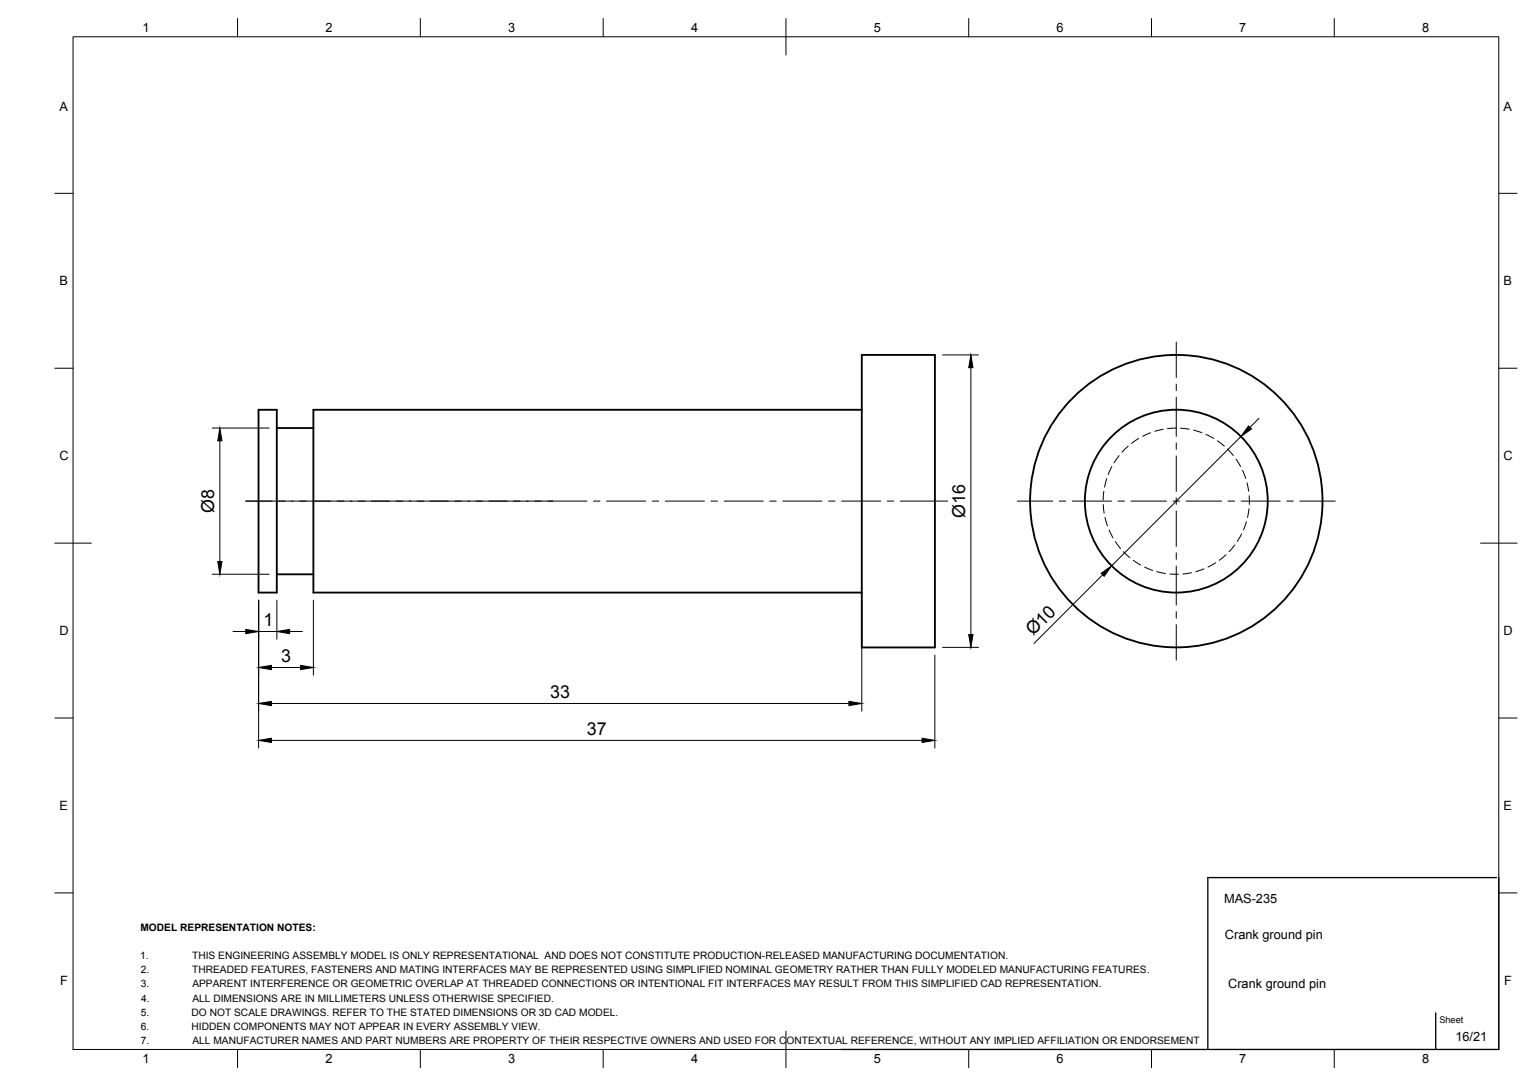
ISO-10303-21;
HEADER;
/* Generated by software containing ST-Developer
 * from STEP Tools, Inc. (www.steptools.com) 
 */

FILE_DESCRIPTION(
/* description */ ('Independent Whitworth quick-return mechanism. Crank radius40, ground-
center spacing80, lever180, connecting rod160, output guide X200. Nomi
nal stroke180 and long/short phase ratio2. Retained guide rods, replac
eable bearing sleeves and captured sliding shoe. No load or production
 rating assigned.'),
/* implementation_level */ '2;1');

FILE_NAME(
/* name */ 'Crank ground pin.step',
/* time_stamp */ '2026-11-09T18:22:56-08:00',
/* author */ (''),
/* organization */ (''),
/* preprocessor_version */ 'ST-DEVELOPER v20.2',
/* originating_system */ 'Autodesk Translation Framework v15.17.0.0',
/* authorisation */ '');

FILE_SCHEMA (('AUTOMOTIVE_DESIGN { 1 0 10303 214 3 1 1 }'));
ENDSEC;

DATA;
#10=MECHANICAL_DESIGN_GEOMETRIC_PRESENTATION_REPRESENTATION('',(#230),#4388);
#190=SHAPE_REPRESENTATION_RELATIONSHIP('SRR','None',#4489,#210);
#210=ADVANCED_BREP_SHAPE_REPRESENTATION('',(#250),#4379);
#230=STYLED_ITEM('',(#4595),#250);
#250=MANIFOLD_SOLID_BREP('Body1',#2335);
#296=FACE_BOUND('',#671,.T.);
#297=FACE_BOUND('',#673,.T.);
#298=FACE_BOUND('',#676,.T.);
#368=PLANE('',#2723);
#369=PLANE('',#2725);
#370=PLANE('',#2729);
#371=PLANE('',#2734);
#372=PLANE('',#2736);
#485=FACE_OUTER_BOUND('',#669,.T.);
#486=FACE_OUTER_BOUND('',#670,.T.);
#487=FACE_OUTER_BOUND('',#672,.T.);
#488=FACE_OUTER_BOUND('',#674,.T.);
#489=FACE_OUTER_BOUND('',#675,.T.);
#490=FACE_OUTER_BOUND('',#677,.T.);
#491=FACE_OUTER_BOUND('',#678,.T.);
#492=FACE_OUTER_BOUND('',#679,.T.);
#493=FACE_OUTER_BOUND('',#680,.T.);
#669=EDGE_LOOP('',(#1924,#1925,#1926,#1927));
#670=EDGE_LOOP('',(#1928));
#671=EDGE_LOOP('',(#1929));
#672=EDGE_LOOP('',(#1930));
#673=EDGE_LOOP('',(#1931));
#674=EDGE_LOOP('',(#1932,#1933,#1934,#1935));
#675=EDGE_LOOP('',(#1936));
#676=EDGE_LOOP('',(#1937));
#677=EDGE_LOOP('',(#1938,#1939,#1940,#1941));
#678=EDGE_LOOP('',(#1942));
#679=EDGE_LOOP('',(#1943,#1944,#1945,#1946));
#680=EDGE_LOOP('',(#1947));
#862=LINE('',#4072,#1001);
#863=LINE('',#4083,#1002);
#864=LINE('',#4091,#1003);
#865=LINE('',#4095,#1004);
#1001=VECTOR('',#3314,4.);
#1002=VECTOR('',#3329,5.);
#1003=VECTOR('',#3338,8.);
#1004=VECTOR('',#3345,5.);
#1099=CIRCLE('',#2721,4.);
#1100=CIRCLE('',#2722,4.);
#1101=CIRCLE('',#2724,5.);
#1102=CIRCLE('',#2726,5.);
#1103=CIRCLE('',#2728,5.);
#1104=CIRCLE('',#2730,8.);
#1105=CIRCLE('',#2731,5.);
#1106=CIRCLE('',#2733,8.);
#1269=VERTEX_POINT('',#4069);
#1270=VERTEX_POINT('',#4071);
#1271=VERTEX_POINT('',#4075);
#1272=VERTEX_POINT('',#4078);
#1273=VERTEX_POINT('',#4081);
#1274=VERTEX_POINT('',#4085);
#1275=VERTEX_POINT('',#4087);
#1276=VERTEX_POINT('',#4090);
#1498=EDGE_CURVE('',#1269,#1269,#1099,.T.);
#1499=EDGE_CURVE('',#1269,#1270,#862,.T.);
#1500=EDGE_CURVE('',#1270,#1270,#1100,.T.);
#1501=EDGE_CURVE('',#1271,#1271,#1101,.T.);
#1502=EDGE_CURVE('',#1272,#1272,#1102,.T.);
#1503=EDGE_CURVE('',#1273,#1273,#1103,.T.);
#1504=EDGE_CURVE('',#1273,#1272,#863,.T.);
#1505=EDGE_CURVE('',#1274,#1274,#1104,.T.);
#1506=EDGE_CURVE('',#1275,#1275,#1105,.T.);
#1507=EDGE_CURVE('',#1274,#1276,#864,.T.);
#1508=EDGE_CURVE('',#1276,#1276,#1106,.T.);
#1509=EDGE_CURVE('',#1271,#1275,#865,.T.);
#1924=ORIENTED_EDGE('',*,*,#1498,.T.);
#1925=ORIENTED_EDGE('',*,*,#1499,.T.);
#1926=ORIENTED_EDGE('',*,*,#1500,.F.);
#1927=ORIENTED_EDGE('',*,*,#1499,.F.);
#1928=ORIENTED_EDGE('',*,*,#1501,.F.);
#1929=ORIENTED_EDGE('',*,*,#1498,.F.);
#1930=ORIENTED_EDGE('',*,*,#1502,.F.);
#1931=ORIENTED_EDGE('',*,*,#1500,.T.);
#1932=ORIENTED_EDGE('',*,*,#1503,.F.);
#1933=ORIENTED_EDGE('',*,*,#1504,.T.);
#1934=ORIENTED_EDGE('',*,*,#1502,.T.);
#1935=ORIENTED_EDGE('',*,*,#1504,.F.);
#1936=ORIENTED_EDGE('',*,*,#1505,.T.);
#1937=ORIENTED_EDGE('',*,*,#1506,.F.);
#1938=ORIENTED_EDGE('',*,*,#1505,.F.);
#1939=ORIENTED_EDGE('',*,*,#1507,.T.);
#1940=ORIENTED_EDGE('',*,*,#1508,.T.);
#1941=ORIENTED_EDGE('',*,*,#1507,.F.);
#1942=ORIENTED_EDGE('',*,*,#1508,.F.);
#1943=ORIENTED_EDGE('',*,*,#1501,.T.);
#1944=ORIENTED_EDGE('',*,*,#1509,.T.);
#1945=ORIENTED_EDGE('',*,*,#1506,.T.);
#1946=ORIENTED_EDGE('',*,*,#1509,.F.);
#1947=ORIENTED_EDGE('',*,*,#1503,.T.);
#2147=CYLINDRICAL_SURFACE('',#2720,4.);
#2148=CYLINDRICAL_SURFACE('',#2727,5.);
#2149=CYLINDRICAL_SURFACE('',#2732,8.);
#2150=CYLINDRICAL_SURFACE('',#2735,5.);
#2257=ADVANCED_FACE('',(#485),#2147,.T.);
#2258=ADVANCED_FACE('',(#486,#296),#368,.F.);
#2259=ADVANCED_FACE('',(#487,#297),#369,.F.);
#2260=ADVANCED_FACE('',(#488),#2148,.T.);
#2261=ADVANCED_FACE('',(#489,#298),#370,.T.);
#2262=ADVANCED_FACE('',(#490),#2149,.T.);
#2263=ADVANCED_FACE('',(#491),#371,.F.);
#2264=ADVANCED_FACE('',(#492),#2150,.T.);
#2265=ADVANCED_FACE('',(#493),#372,.T.);
#2335=CLOSED_SHELL('',(#2257,#2258,#2259,#2260,#2261,#2262,#2263,#2264,
#2265));
#2719=AXIS2_PLACEMENT_3D('',#4067,#3308,#3309);
#2720=AXIS2_PLACEMENT_3D('',#4068,#3310,#3311);
#2721=AXIS2_PLACEMENT_3D('',#4070,#3312,#3313);
#2722=AXIS2_PLACEMENT_3D('',#4073,#3315,#3316);
#2723=AXIS2_PLACEMENT_3D('',#4074,#3317,#3318);
#2724=AXIS2_PLACEMENT_3D('',#4076,#3319,#3320);
#2725=AXIS2_PLACEMENT_3D('',#4077,#3321,#3322);
#2726=AXIS2_PLACEMENT_3D('',#4079,#3323,#3324);
#2727=AXIS2_PLACEMENT_3D('',#4080,#3325,#3326);
#2728=AXIS2_PLACEMENT_3D('',#4082,#3327,#3328);
#2729=AXIS2_PLACEMENT_3D('',#4084,#3330,#3331);
#2730=AXIS2_PLACEMENT_3D('',#4086,#3332,#3333);
#2731=AXIS2_PLACEMENT_3D('',#4088,#3334,#3335);
#2732=AXIS2_PLACEMENT_3D('',#4089,#3336,#3337);
#2733=AXIS2_PLACEMENT_3D('',#4092,#3339,#3340);
#2734=AXIS2_PLACEMENT_3D('',#4093,#3341,#3342);
#2735=AXIS2_PLACEMENT_3D('',#4094,#3343,#3344);
#2736=AXIS2_PLACEMENT_3D('',#4096,#3346,#3347);
#3308=DIRECTION('axis',(0.,0.,1.));
#3309=DIRECTION('refdir',(1.,0.,0.));
#3310=DIRECTION('center_axis',(0.,0.,1.));
#3311=DIRECTION('ref_axis',(1.,0.,0.));
#3312=DIRECTION('center_axis',(0.,0.,1.));
#3313=DIRECTION('ref_axis',(1.,0.,0.));
#3314=DIRECTION('',(0.,0.,1.));
#3315=DIRECTION('center_axis',(0.,0.,1.));
#3316=DIRECTION('ref_axis',(1.,0.,0.));
#3317=DIRECTION('center_axis',(0.,0.,-1.));
#3318=DIRECTION('ref_axis',(-1.,0.,0.));
#3319=DIRECTION('center_axis',(0.,0.,-1.));
#3320=DIRECTION('ref_axis',(1.,0.,0.));
#3321=DIRECTION('center_axis',(0.,0.,1.));
#3322=DIRECTION('ref_axis',(1.,0.,0.));
#3323=DIRECTION('center_axis',(0.,0.,1.));
#3324=DIRECTION('ref_axis',(1.,0.,0.));
#3325=DIRECTION('center_axis',(0.,0.,1.));
#3326=DIRECTION('ref_axis',(1.,0.,0.));
#3327=DIRECTION('center_axis',(0.,0.,1.));
#3328=DIRECTION('ref_axis',(1.,0.,0.));
#3329=DIRECTION('',(0.,0.,-1.));
#3330=DIRECTION('center_axis',(0.,0.,1.));
#3331=DIRECTION('ref_axis',(1.,0.,0.));
#3332=DIRECTION('center_axis',(0.,0.,1.));
#3333=DIRECTION('ref_axis',(1.,0.,0.));
#3334=DIRECTION('center_axis',(0.,0.,1.));
#3335=DIRECTION('ref_axis',(1.,0.,0.));
#3336=DIRECTION('center_axis',(0.,0.,1.));
#3337=DIRECTION('ref_axis',(1.,0.,0.));
#3338=DIRECTION('',(0.,0.,-1.));
#3339=DIRECTION('center_axis',(0.,0.,1.));
#3340=DIRECTION('ref_axis',(1.,0.,0.));
#3341=DIRECTION('center_axis',(0.,0.,1.));
#3342=DIRECTION('ref_axis',(1.,0.,0.));
#3343=DIRECTION('center_axis',(0.,0.,1.));
#3344=DIRECTION('ref_axis',(1.,0.,0.));
#3345=DIRECTION('',(0.,0.,-1.));
#3346=DIRECTION('center_axis',(0.,0.,1.));
#3347=DIRECTION('ref_axis',(1.,0.,0.));
#4067=CARTESIAN_POINT('',(0.,0.,0.));
#4068=CARTESIAN_POINT('Origin',(0.,0.,31.));
#4069=CARTESIAN_POINT('',(-4.,-4.89858719658941E-16,30.));
#4070=CARTESIAN_POINT('Origin',(0.,0.,30.));
#4071=CARTESIAN_POINT('',(-4.,-4.89858719658941E-16,32.));
#4072=CARTESIAN_POINT('',(-4.,-4.89858719658941E-16,31.));
#4073=CARTESIAN_POINT('Origin',(0.,0.,32.));
#4074=CARTESIAN_POINT('Origin',(8.,0.,30.));
#4075=CARTESIAN_POINT('',(-5.,6.12323399573677E-16,30.));
#4076=CARTESIAN_POINT('Origin',(0.,0.,30.));
#4077=CARTESIAN_POINT('Origin',(4.,0.,32.));
#4078=CARTESIAN_POINT('',(-5.,-6.12323399573677E-16,32.));
#4079=CARTESIAN_POINT('Origin',(0.,0.,32.));
#4080=CARTESIAN_POINT('Origin',(0.,0.,0.));
#4081=CARTESIAN_POINT('',(-5.,-6.12323399573677E-16,33.));
#4082=CARTESIAN_POINT('Origin',(0.,0.,33.));
#4083=CARTESIAN_POINT('',(-5.,-6.12323399573677E-16,0.));
#4084=CARTESIAN_POINT('Origin',(0.,0.,0.));
#4085=CARTESIAN_POINT('',(-8.,-9.79717439317883E-16,0.));
#4086=CARTESIAN_POINT('Origin',(0.,0.,0.));
#4087=CARTESIAN_POINT('',(-5.,-6.12323399573677E-16,0.));
#4088=CARTESIAN_POINT('Origin',(0.,0.,0.));
#4089=CARTESIAN_POINT('Origin',(0.,0.,-4.));
#4090=CARTESIAN_POINT('',(-8.,-9.79717439317883E-16,-4.));
#4091=CARTESIAN_POINT('',(-8.,-9.79717439317883E-16,-4.));
#4092=CARTESIAN_POINT('Origin',(0.,0.,-4.));
#4093=CARTESIAN_POINT('Origin',(0.,0.,-4.));
#4094=CARTESIAN_POINT('Origin',(0.,0.,0.));
#4095=CARTESIAN_POINT('',(-5.,-6.12323399573677E-16,0.));
#4096=CARTESIAN_POINT('Origin',(0.,0.,33.));
#4357=UNCERTAINTY_MEASURE_WITH_UNIT(LENGTH_MEASURE(0.01),#4389,
'DISTANCE_ACCURACY_VALUE',
'Maximum model space distance between geometric entities at asserted c
onnectivities');
#4366=UNCERTAINTY_MEASURE_WITH_UNIT(LENGTH_MEASURE(0.01),#4389,
'DISTANCE_ACCURACY_VALUE',
'Maximum model space distance between geometric entities at asserted c
onnectivities');
#4379=(
GEOMETRIC_REPRESENTATION_CONTEXT(3)
GLOBAL_UNCERTAINTY_ASSIGNED_CONTEXT((#4357))
GLOBAL_UNIT_ASSIGNED_CONTEXT((#4389,#4391,#4392))
REPRESENTATION_CONTEXT('','3D')
);
#4388=(
GEOMETRIC_REPRESENTATION_CONTEXT(3)
GLOBAL_UNCERTAINTY_ASSIGNED_CONTEXT((#4366))
GLOBAL_UNIT_ASSIGNED_CONTEXT((#4389,#4391,#4392))
REPRESENTATION_CONTEXT('','3D')
);
#4389=(
LENGTH_UNIT()
NAMED_UNIT(*)
SI_UNIT(.MILLI.,.METRE.)
);
#4391=(
NAMED_UNIT(*)
PLANE_ANGLE_UNIT()
SI_UNIT($,.RADIAN.)
);
#4392=(
NAMED_UNIT(*)
SI_UNIT($,.STERADIAN.)
SOLID_ANGLE_UNIT()
);
#4405=SHAPE_DEFINITION_REPRESENTATION(#4426,#4489);
#4426=PRODUCT_DEFINITION_SHAPE('',$,#4511);
#4489=SHAPE_REPRESENTATION('',(#2719),#4379);
#4498=PRODUCT_DEFINITION_CONTEXT('part definition',#4563,'design');
#4511=PRODUCT_DEFINITION('Crank ground pin','Crank ground pin',#4532,#4498);
#4532=PRODUCT_DEFINITION_FORMATION('',$,#4577);
#4563=APPLICATION_CONTEXT(
'Core Data for Automotive Mechanical Design Process');
#4564=PRODUCT_CONTEXT('part definition',#4563,'mechanical');
#4577=PRODUCT('Crank ground pin','Crank ground pin',$,(#4564));
#4595=PRESENTATION_STYLE_ASSIGNMENT((#4609));
#4609=SURFACE_STYLE_USAGE(.BOTH.,#4623);
#4623=SURFACE_SIDE_STYLE('',(#4637));
#4637=SURFACE_STYLE_FILL_AREA(#4651);
#4651=FILL_AREA_STYLE('Pivot gray',(#4665));
#4665=FILL_AREA_STYLE_COLOUR('Pivot gray',#4679);
#4679=COLOUR_RGB('Pivot gray',0.407843137254902,0.447058823529412,0.498039215686275);
ENDSEC;
END-ISO-10303-21;
